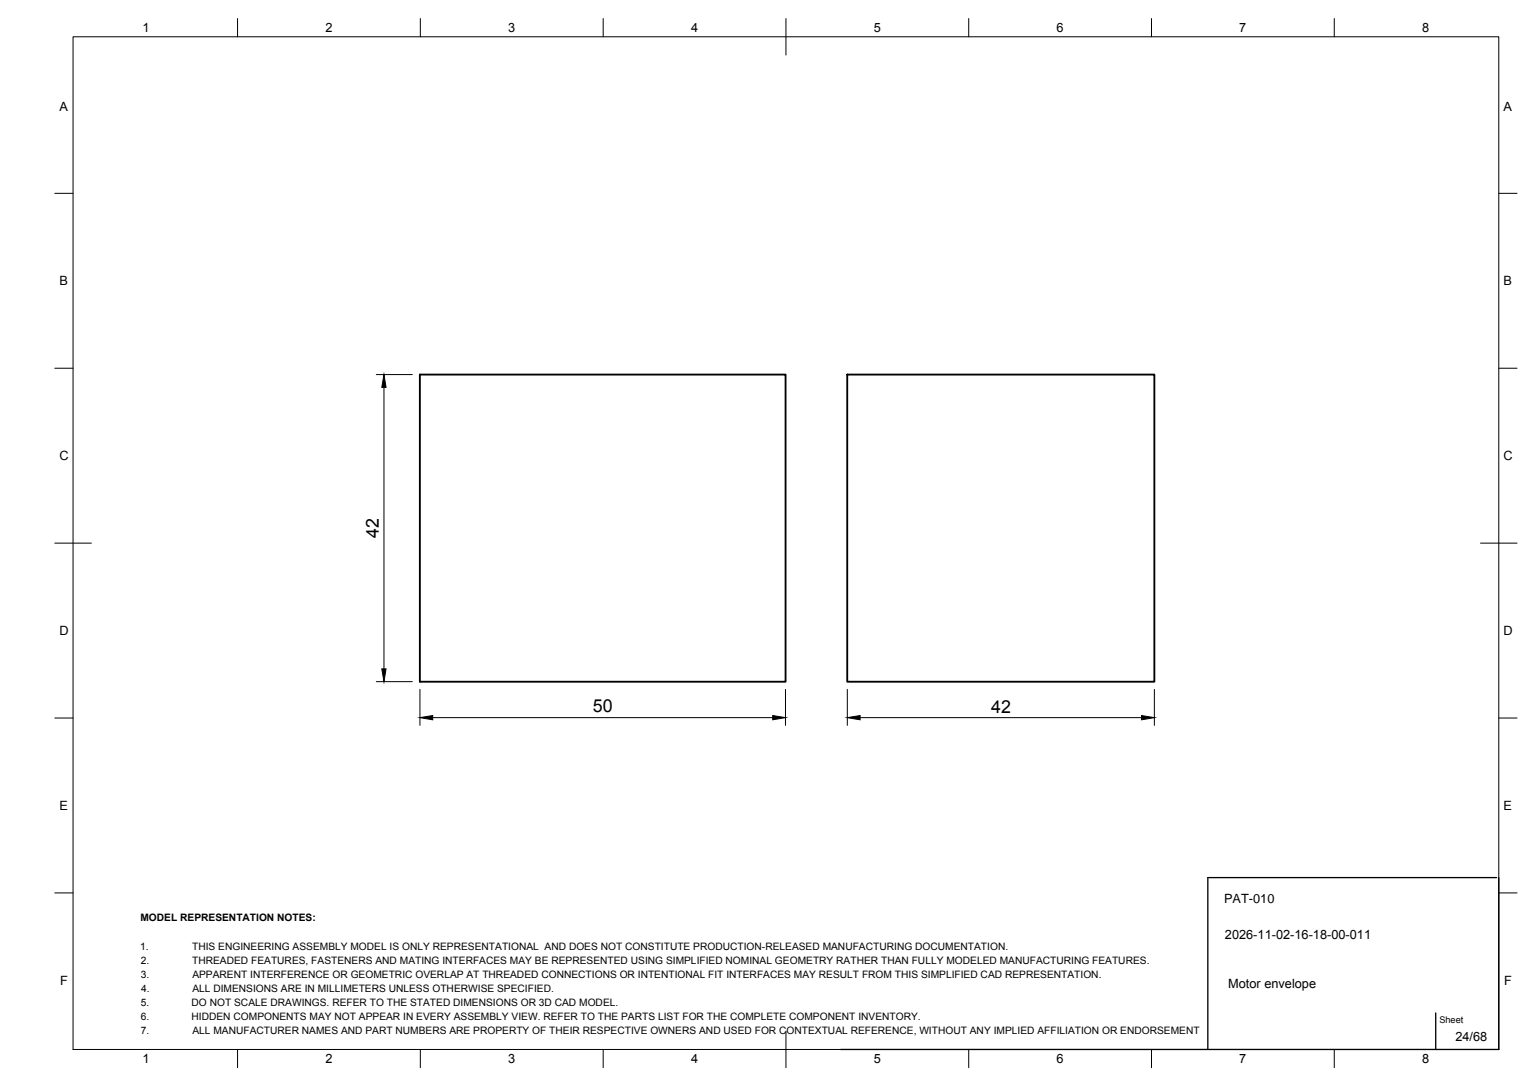
ISO-10303-21;
HEADER;
/* Generated by software containing ST-Developer
 * from STEP Tools, Inc. (www.steptools.com) 
 */

FILE_DESCRIPTION(
/* description */ ('Belt conveyor head drive unit'),
/* implementation_level */ '2;1');

FILE_NAME(
/* name */ 'Motor envelope.step',
/* time_stamp */ '2026-10-28T03:26:19-07:00',
/* author */ (''),
/* organization */ (''),
/* preprocessor_version */ 'ST-DEVELOPER v20.2',
/* originating_system */ 'Autodesk Translation Framework v15.17.0.0',
/* authorisation */ '');

FILE_SCHEMA (('AUTOMOTIVE_DESIGN { 1 0 10303 214 3 1 1 }'));
ENDSEC;

DATA;
#10=MECHANICAL_DESIGN_GEOMETRIC_PRESENTATION_REPRESENTATION('',(#870),#27069);
#732=SHAPE_REPRESENTATION_RELATIONSHIP('SRR','None',#27376,#801);
#801=ADVANCED_BREP_SHAPE_REPRESENTATION('',(#955),#27018);
#870=STYLED_ITEM('',(#27790),#955);
#955=MANIFOLD_SOLID_BREP('Body1',#13735);
#1413=PLANE('',#15138);
#1414=PLANE('',#15139);
#1415=PLANE('',#15140);
#1416=PLANE('',#15141);
#1417=PLANE('',#15142);
#1418=PLANE('',#15143);
#1903=FACE_OUTER_BOUND('',#2826,.T.);
#1904=FACE_OUTER_BOUND('',#2827,.T.);
#1905=FACE_OUTER_BOUND('',#2828,.T.);
#1906=FACE_OUTER_BOUND('',#2829,.T.);
#1907=FACE_OUTER_BOUND('',#2830,.T.);
#1908=FACE_OUTER_BOUND('',#2831,.T.);
#2826=EDGE_LOOP('',(#10128,#10129,#10130,#10131));
#2827=EDGE_LOOP('',(#10132,#10133,#10134,#10135));
#2828=EDGE_LOOP('',(#10136,#10137,#10138,#10139));
#2829=EDGE_LOOP('',(#10140,#10141,#10142,#10143));
#2830=EDGE_LOOP('',(#10144,#10145,#10146,#10147));
#2831=EDGE_LOOP('',(#10148,#10149,#10150,#10151));
#3803=LINE('',#22244,#4595);
#3804=LINE('',#22246,#4596);
#3805=LINE('',#22248,#4597);
#3806=LINE('',#22249,#4598);
#3807=LINE('',#22252,#4599);
#3808=LINE('',#22254,#4600);
#3809=LINE('',#22255,#4601);
#3810=LINE('',#22258,#4602);
#3811=LINE('',#22260,#4603);
#3812=LINE('',#22261,#4604);
#3813=LINE('',#22263,#4605);
#3814=LINE('',#22264,#4606);
#4595=VECTOR('',#17893,1.);
#4596=VECTOR('',#17894,1.);
#4597=VECTOR('',#17895,1.);
#4598=VECTOR('',#17896,1.);
#4599=VECTOR('',#17899,1.);
#4600=VECTOR('',#17900,1.);
#4601=VECTOR('',#17901,1.);
#4602=VECTOR('',#17904,1.);
#4603=VECTOR('',#17905,1.);
#4604=VECTOR('',#17906,1.);
#4605=VECTOR('',#17909,1.);
#4606=VECTOR('',#17910,1.);
#6343=VERTEX_POINT('',#22242);
#6344=VERTEX_POINT('',#22243);
#6345=VERTEX_POINT('',#22245);
#6346=VERTEX_POINT('',#22247);
#6347=VERTEX_POINT('',#22251);
#6348=VERTEX_POINT('',#22253);
#6349=VERTEX_POINT('',#22257);
#6350=VERTEX_POINT('',#22259);
#7756=EDGE_CURVE('',#6343,#6344,#3803,.T.);
#7757=EDGE_CURVE('',#6344,#6345,#3804,.T.);
#7758=EDGE_CURVE('',#6346,#6345,#3805,.T.);
#7759=EDGE_CURVE('',#6343,#6346,#3806,.T.);
#7760=EDGE_CURVE('',#6347,#6343,#3807,.T.);
#7761=EDGE_CURVE('',#6348,#6346,#3808,.T.);
#7762=EDGE_CURVE('',#6347,#6348,#3809,.T.);
#7763=EDGE_CURVE('',#6349,#6347,#3810,.T.);
#7764=EDGE_CURVE('',#6350,#6348,#3811,.T.);
#7765=EDGE_CURVE('',#6349,#6350,#3812,.T.);
#7766=EDGE_CURVE('',#6344,#6349,#3813,.T.);
#7767=EDGE_CURVE('',#6345,#6350,#3814,.T.);
#10128=ORIENTED_EDGE('',*,*,#7756,.T.);
#10129=ORIENTED_EDGE('',*,*,#7757,.T.);
#10130=ORIENTED_EDGE('',*,*,#7758,.F.);
#10131=ORIENTED_EDGE('',*,*,#7759,.F.);
#10132=ORIENTED_EDGE('',*,*,#7760,.T.);
#10133=ORIENTED_EDGE('',*,*,#7759,.T.);
#10134=ORIENTED_EDGE('',*,*,#7761,.F.);
#10135=ORIENTED_EDGE('',*,*,#7762,.F.);
#10136=ORIENTED_EDGE('',*,*,#7763,.T.);
#10137=ORIENTED_EDGE('',*,*,#7762,.T.);
#10138=ORIENTED_EDGE('',*,*,#7764,.F.);
#10139=ORIENTED_EDGE('',*,*,#7765,.F.);
#10140=ORIENTED_EDGE('',*,*,#7766,.T.);
#10141=ORIENTED_EDGE('',*,*,#7765,.T.);
#10142=ORIENTED_EDGE('',*,*,#7767,.F.);
#10143=ORIENTED_EDGE('',*,*,#7757,.F.);
#10144=ORIENTED_EDGE('',*,*,#7767,.T.);
#10145=ORIENTED_EDGE('',*,*,#7764,.T.);
#10146=ORIENTED_EDGE('',*,*,#7761,.T.);
#10147=ORIENTED_EDGE('',*,*,#7758,.T.);
#10148=ORIENTED_EDGE('',*,*,#7766,.F.);
#10149=ORIENTED_EDGE('',*,*,#7756,.F.);
#10150=ORIENTED_EDGE('',*,*,#7760,.F.);
#10151=ORIENTED_EDGE('',*,*,#7763,.F.);
#13182=ADVANCED_FACE('',(#1903),#1413,.T.);
#13183=ADVANCED_FACE('',(#1904),#1414,.T.);
#13184=ADVANCED_FACE('',(#1905),#1415,.T.);
#13185=ADVANCED_FACE('',(#1906),#1416,.T.);
#13186=ADVANCED_FACE('',(#1907),#1417,.T.);
#13187=ADVANCED_FACE('',(#1908),#1418,.F.);
#13735=CLOSED_SHELL('',(#13182,#13183,#13184,#13185,#13186,#13187));
#15137=AXIS2_PLACEMENT_3D('',#22240,#17889,#17890);
#15138=AXIS2_PLACEMENT_3D('',#22241,#17891,#17892);
#15139=AXIS2_PLACEMENT_3D('',#22250,#17897,#17898);
#15140=AXIS2_PLACEMENT_3D('',#22256,#17902,#17903);
#15141=AXIS2_PLACEMENT_3D('',#22262,#17907,#17908);
#15142=AXIS2_PLACEMENT_3D('',#22265,#17911,#17912);
#15143=AXIS2_PLACEMENT_3D('',#22266,#17913,#17914);
#17889=DIRECTION('axis',(0.,0.,1.));
#17890=DIRECTION('refdir',(1.,0.,0.));
#17891=DIRECTION('center_axis',(0.,1.,0.));
#17892=DIRECTION('ref_axis',(-1.,0.,0.));
#17893=DIRECTION('',(-1.,0.,0.));
#17894=DIRECTION('',(0.,0.,1.));
#17895=DIRECTION('',(-1.,0.,0.));
#17896=DIRECTION('',(0.,0.,1.));
#17897=DIRECTION('center_axis',(1.,0.,0.));
#17898=DIRECTION('ref_axis',(0.,1.,0.));
#17899=DIRECTION('',(0.,1.,0.));
#17900=DIRECTION('',(0.,1.,0.));
#17901=DIRECTION('',(0.,0.,1.));
#17902=DIRECTION('center_axis',(0.,-1.,0.));
#17903=DIRECTION('ref_axis',(1.,0.,0.));
#17904=DIRECTION('',(1.,0.,0.));
#17905=DIRECTION('',(1.,0.,0.));
#17906=DIRECTION('',(0.,0.,1.));
#17907=DIRECTION('center_axis',(-1.,0.,0.));
#17908=DIRECTION('ref_axis',(0.,-1.,0.));
#17909=DIRECTION('',(0.,-1.,0.));
#17910=DIRECTION('',(0.,-1.,0.));
#17911=DIRECTION('center_axis',(0.,0.,1.));
#17912=DIRECTION('ref_axis',(1.,0.,0.));
#17913=DIRECTION('center_axis',(0.,0.,1.));
#17914=DIRECTION('ref_axis',(1.,0.,0.));
#22240=CARTESIAN_POINT('',(0.,0.,0.));
#22241=CARTESIAN_POINT('Origin',(2.1,10.,4.9));
#22242=CARTESIAN_POINT('',(2.1,10.,4.9));
#22243=CARTESIAN_POINT('',(-2.1,10.,4.9));
#22244=CARTESIAN_POINT('',(2.1,10.,4.9));
#22245=CARTESIAN_POINT('',(-2.1,10.,9.1));
#22246=CARTESIAN_POINT('',(-2.1,10.,4.9));
#22247=CARTESIAN_POINT('',(2.1,10.,9.1));
#22248=CARTESIAN_POINT('',(2.1,10.,9.1));
#22249=CARTESIAN_POINT('',(2.1,10.,4.9));
#22250=CARTESIAN_POINT('Origin',(2.1,5.,4.9));
#22251=CARTESIAN_POINT('',(2.1,5.,4.9));
#22252=CARTESIAN_POINT('',(2.1,5.,4.9));
#22253=CARTESIAN_POINT('',(2.1,5.,9.1));
#22254=CARTESIAN_POINT('',(2.1,5.,9.1));
#22255=CARTESIAN_POINT('',(2.1,5.,4.9));
#22256=CARTESIAN_POINT('Origin',(-2.1,5.,4.9));
#22257=CARTESIAN_POINT('',(-2.1,5.,4.9));
#22258=CARTESIAN_POINT('',(-2.1,5.,4.9));
#22259=CARTESIAN_POINT('',(-2.1,5.,9.1));
#22260=CARTESIAN_POINT('',(-2.1,5.,9.1));
#22261=CARTESIAN_POINT('',(-2.1,5.,4.9));
#22262=CARTESIAN_POINT('Origin',(-2.1,10.,4.9));
#22263=CARTESIAN_POINT('',(-2.1,10.,4.9));
#22264=CARTESIAN_POINT('',(-2.1,10.,9.1));
#22265=CARTESIAN_POINT('Origin',(0.,7.5,9.1));
#22266=CARTESIAN_POINT('Origin',(0.,7.5,4.9));
#26941=UNCERTAINTY_MEASURE_WITH_UNIT(LENGTH_MEASURE(0.001),#27070,
'DISTANCE_ACCURACY_VALUE',
'Maximum model space distance between geometric entities at asserted c
onnectivities');
#26992=UNCERTAINTY_MEASURE_WITH_UNIT(LENGTH_MEASURE(0.001),#27070,
'DISTANCE_ACCURACY_VALUE',
'Maximum model space distance between geometric entities at asserted c
onnectivities');
#27018=(
GEOMETRIC_REPRESENTATION_CONTEXT(3)
GLOBAL_UNCERTAINTY_ASSIGNED_CONTEXT((#26941))
GLOBAL_UNIT_ASSIGNED_CONTEXT((#27070,#27072,#27073))
REPRESENTATION_CONTEXT('','3D')
);
#27069=(
GEOMETRIC_REPRESENTATION_CONTEXT(3)
GLOBAL_UNCERTAINTY_ASSIGNED_CONTEXT((#26992))
GLOBAL_UNIT_ASSIGNED_CONTEXT((#27070,#27072,#27073))
REPRESENTATION_CONTEXT('','3D')
);
#27070=(
LENGTH_UNIT()
NAMED_UNIT(*)
SI_UNIT(.CENTI.,.METRE.)
);
#27072=(
NAMED_UNIT(*)
PLANE_ANGLE_UNIT()
SI_UNIT($,.RADIAN.)
);
#27073=(
NAMED_UNIT(*)
SI_UNIT($,.STERADIAN.)
SOLID_ANGLE_UNIT()
);
#27099=SHAPE_DEFINITION_REPRESENTATION(#27175,#27376);
#27175=PRODUCT_DEFINITION_SHAPE('',$,#27453);
#27376=SHAPE_REPRESENTATION('',(#15137),#27018);
#27427=PRODUCT_DEFINITION_CONTEXT('part definition',#27657,'design');
#27453=PRODUCT_DEFINITION('Motor envelope','Motor envelope',#27529,#27427);
#27529=PRODUCT_DEFINITION_FORMATION('',$,#27684);
#27657=APPLICATION_CONTEXT(
'Core Data for Automotive Mechanical Design Process');
#27658=PRODUCT_CONTEXT('part definition',#27657,'mechanical');
#27684=PRODUCT('Motor envelope','Motor envelope','Motor envelope',(#27658));
#27784=COLOUR_RGB('Sky Blue',0.24,0.69,0.87);
#27785=FILL_AREA_STYLE_COLOUR('',#27784);
#27786=FILL_AREA_STYLE('',(#27785));
#27787=SURFACE_STYLE_FILL_AREA(#27786);
#27788=SURFACE_SIDE_STYLE('',(#27787));
#27789=SURFACE_STYLE_USAGE(.BOTH.,#27788);
#27790=PRESENTATION_STYLE_ASSIGNMENT((#27789));
ENDSEC;
END-ISO-10303-21;
